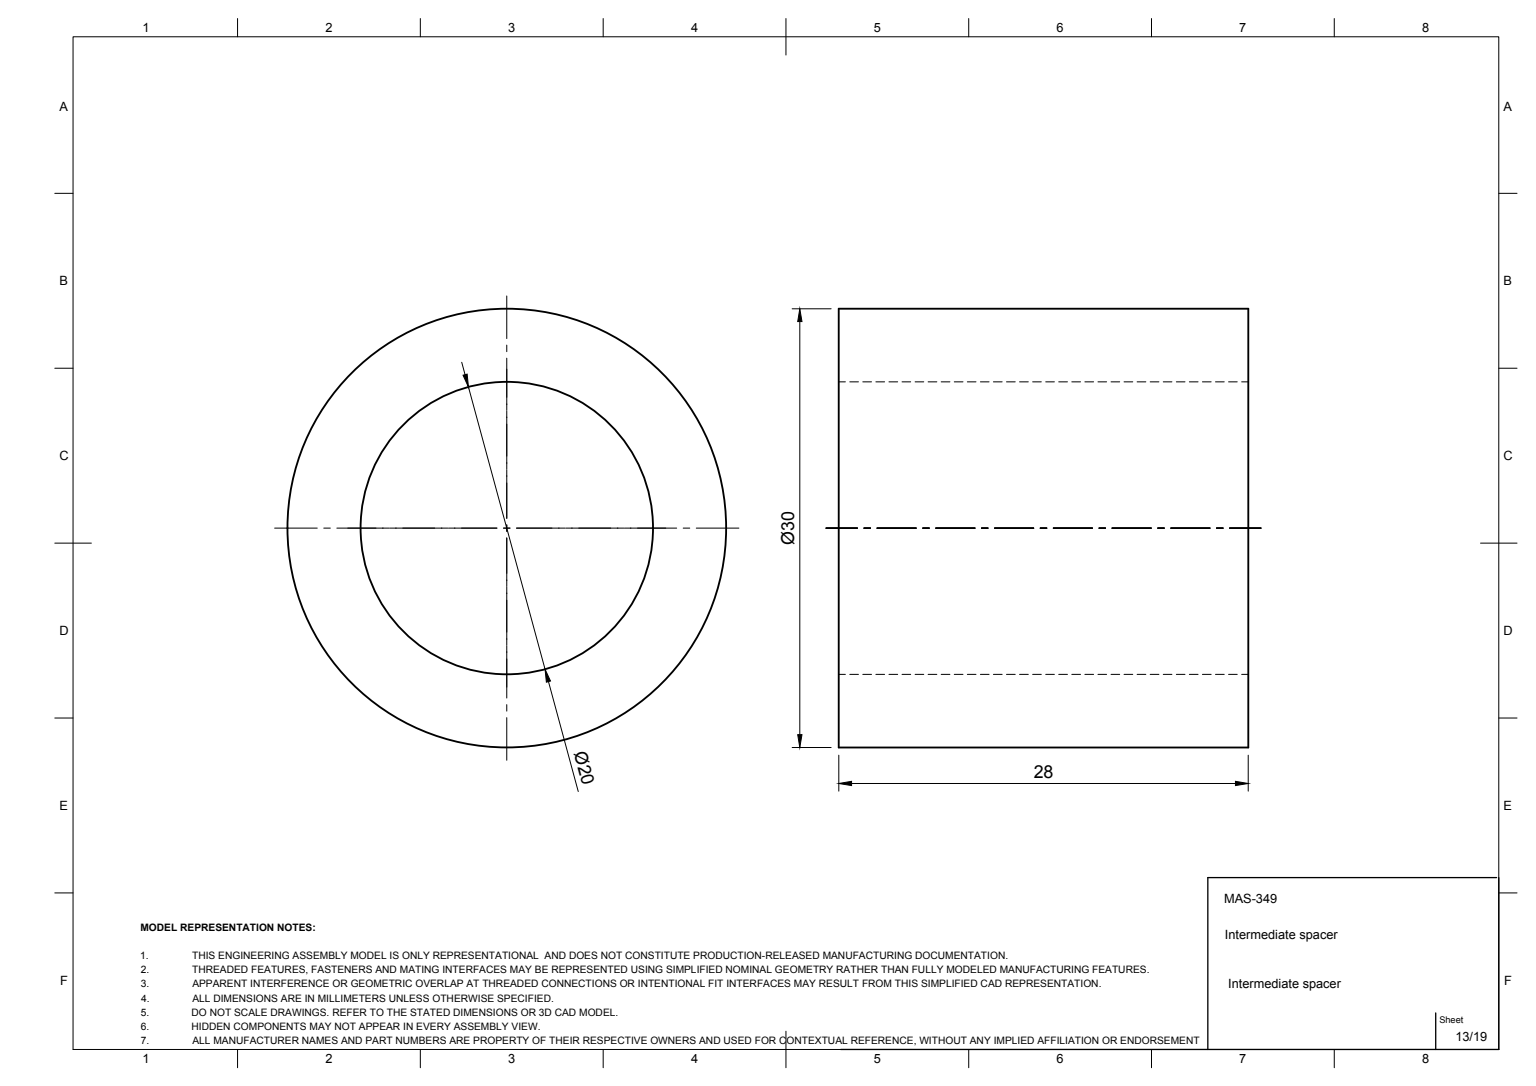
ISO-10303-21;
HEADER;
/* Generated by software containing ST-Developer
 * from STEP Tools, Inc. (www.steptools.com) 
 */

FILE_DESCRIPTION(
/* description */ ('Independent two-stage semi-open centrifugal-pump CAD. Shared impeller
s, open-machinable return casings, removable diaphragms, bronze wear/j
ournal rings, volume-preserving seal instances, retained keyed shaft, 
opposed mechanical face rings and partly threaded tie hardware. Native
 shaft rotation. Geometric topology/clearance only; flow/head/efficien
cy, pressure, cavitation, balance, preload, face loading and secondary
 seal fits/bonds, material/thermal/tolerance selection and life unassi
gned. External drive, coupling, anchors and piping bolts omitted.'),
/* implementation_level */ '2;1');

FILE_NAME(
/* name */ 'Intermediate spacer.step',
/* time_stamp */ '2026-11-08T18:06:32-08:00',
/* author */ (''),
/* organization */ (''),
/* preprocessor_version */ 'ST-DEVELOPER v20.2',
/* originating_system */ 'Autodesk Translation Framework v15.17.0.0',
/* authorisation */ '');

FILE_SCHEMA (('AUTOMOTIVE_DESIGN { 1 0 10303 214 3 1 1 }'));
ENDSEC;

DATA;
#10=MECHANICAL_DESIGN_GEOMETRIC_PRESENTATION_REPRESENTATION('',(#402),#16687);
#364=SHAPE_REPRESENTATION_RELATIONSHIP('SRR','None',#16773,#383);
#383=ADVANCED_BREP_SHAPE_REPRESENTATION('',(#421),#16677);
#402=STYLED_ITEM('',(#16874),#421);
#421=MANIFOLD_SOLID_BREP('Body1',#6121);
#537=FACE_BOUND('',#1418,.T.);
#538=FACE_BOUND('',#1420,.T.);
#653=PLANE('',#6840);
#654=PLANE('',#6841);
#962=FACE_OUTER_BOUND('',#1415,.T.);
#963=FACE_OUTER_BOUND('',#1416,.T.);
#964=FACE_OUTER_BOUND('',#1417,.T.);
#965=FACE_OUTER_BOUND('',#1419,.T.);
#1415=EDGE_LOOP('',(#5269,#5270,#5271,#5272));
#1416=EDGE_LOOP('',(#5273,#5274,#5275,#5276));
#1417=EDGE_LOOP('',(#5277));
#1418=EDGE_LOOP('',(#5278));
#1419=EDGE_LOOP('',(#5279));
#1420=EDGE_LOOP('',(#5280));
#1806=LINE('',#15120,#2175);
#1807=LINE('',#15126,#2176);
#2175=VECTOR('',#8282,1.);
#2176=VECTOR('',#8289,1.5);
#2454=CIRCLE('',#6835,1.);
#2455=CIRCLE('',#6836,1.);
#2456=CIRCLE('',#6838,1.5);
#2457=CIRCLE('',#6839,1.5);
#2957=VERTEX_POINT('',#15117);
#2958=VERTEX_POINT('',#15119);
#2959=VERTEX_POINT('',#15123);
#2960=VERTEX_POINT('',#15125);
#3744=EDGE_CURVE('',#2957,#2957,#2454,.T.);
#3745=EDGE_CURVE('',#2957,#2958,#1806,.T.);
#3746=EDGE_CURVE('',#2958,#2958,#2455,.T.);
#3747=EDGE_CURVE('',#2959,#2959,#2456,.T.);
#3748=EDGE_CURVE('',#2959,#2960,#1807,.T.);
#3749=EDGE_CURVE('',#2960,#2960,#2457,.T.);
#5269=ORIENTED_EDGE('',*,*,#3744,.F.);
#5270=ORIENTED_EDGE('',*,*,#3745,.T.);
#5271=ORIENTED_EDGE('',*,*,#3746,.T.);
#5272=ORIENTED_EDGE('',*,*,#3745,.F.);
#5273=ORIENTED_EDGE('',*,*,#3747,.F.);
#5274=ORIENTED_EDGE('',*,*,#3748,.T.);
#5275=ORIENTED_EDGE('',*,*,#3749,.T.);
#5276=ORIENTED_EDGE('',*,*,#3748,.F.);
#5277=ORIENTED_EDGE('',*,*,#3747,.T.);
#5278=ORIENTED_EDGE('',*,*,#3744,.T.);
#5279=ORIENTED_EDGE('',*,*,#3749,.F.);
#5280=ORIENTED_EDGE('',*,*,#3746,.F.);
#5730=CYLINDRICAL_SURFACE('',#6834,1.);
#5731=CYLINDRICAL_SURFACE('',#6837,1.5);
#6041=ADVANCED_FACE('',(#962),#5730,.F.);
#6042=ADVANCED_FACE('',(#963),#5731,.T.);
#6043=ADVANCED_FACE('',(#964,#537),#653,.T.);
#6044=ADVANCED_FACE('',(#965,#538),#654,.F.);
#6121=CLOSED_SHELL('',(#6041,#6042,#6043,#6044));
#6833=AXIS2_PLACEMENT_3D('',#15115,#8276,#8277);
#6834=AXIS2_PLACEMENT_3D('',#15116,#8278,#8279);
#6835=AXIS2_PLACEMENT_3D('',#15118,#8280,#8281);
#6836=AXIS2_PLACEMENT_3D('',#15121,#8283,#8284);
#6837=AXIS2_PLACEMENT_3D('',#15122,#8285,#8286);
#6838=AXIS2_PLACEMENT_3D('',#15124,#8287,#8288);
#6839=AXIS2_PLACEMENT_3D('',#15127,#8290,#8291);
#6840=AXIS2_PLACEMENT_3D('',#15128,#8292,#8293);
#6841=AXIS2_PLACEMENT_3D('',#15129,#8294,#8295);
#8276=DIRECTION('axis',(0.,0.,1.));
#8277=DIRECTION('refdir',(1.,0.,0.));
#8278=DIRECTION('center_axis',(0.,0.,1.));
#8279=DIRECTION('ref_axis',(1.,0.,0.));
#8280=DIRECTION('center_axis',(0.,0.,-1.));
#8281=DIRECTION('ref_axis',(1.,0.,0.));
#8282=DIRECTION('',(0.,0.,-1.));
#8283=DIRECTION('center_axis',(0.,0.,-1.));
#8284=DIRECTION('ref_axis',(1.,0.,0.));
#8285=DIRECTION('center_axis',(0.,0.,1.));
#8286=DIRECTION('ref_axis',(1.,0.,0.));
#8287=DIRECTION('center_axis',(0.,0.,1.));
#8288=DIRECTION('ref_axis',(1.,0.,0.));
#8289=DIRECTION('',(0.,0.,-1.));
#8290=DIRECTION('center_axis',(0.,0.,1.));
#8291=DIRECTION('ref_axis',(1.,0.,0.));
#8292=DIRECTION('center_axis',(0.,0.,1.));
#8293=DIRECTION('ref_axis',(1.,0.,0.));
#8294=DIRECTION('center_axis',(0.,0.,1.));
#8295=DIRECTION('ref_axis',(1.,0.,0.));
#15115=CARTESIAN_POINT('',(0.,0.,0.));
#15116=CARTESIAN_POINT('Origin',(0.,0.,3.2));
#15117=CARTESIAN_POINT('',(-1.,-1.22464679914735E-16,6.));
#15118=CARTESIAN_POINT('Origin',(0.,0.,6.));
#15119=CARTESIAN_POINT('',(-1.,-1.22464679914735E-16,3.2));
#15120=CARTESIAN_POINT('',(-1.,-1.22464679914735E-16,3.2));
#15121=CARTESIAN_POINT('Origin',(0.,0.,3.2));
#15122=CARTESIAN_POINT('Origin',(0.,0.,3.2));
#15123=CARTESIAN_POINT('',(-1.5,-1.83697019872103E-16,6.));
#15124=CARTESIAN_POINT('Origin',(0.,0.,6.));
#15125=CARTESIAN_POINT('',(-1.5,-1.83697019872103E-16,3.2));
#15126=CARTESIAN_POINT('',(-1.5,-1.83697019872103E-16,3.2));
#15127=CARTESIAN_POINT('Origin',(0.,0.,3.2));
#15128=CARTESIAN_POINT('Origin',(0.,0.,6.));
#15129=CARTESIAN_POINT('Origin',(0.,0.,3.2));
#16656=UNCERTAINTY_MEASURE_WITH_UNIT(LENGTH_MEASURE(0.001),#16688,
'DISTANCE_ACCURACY_VALUE',
'Maximum model space distance between geometric entities at asserted c
onnectivities');
#16666=UNCERTAINTY_MEASURE_WITH_UNIT(LENGTH_MEASURE(0.001),#16688,
'DISTANCE_ACCURACY_VALUE',
'Maximum model space distance between geometric entities at asserted c
onnectivities');
#16677=(
GEOMETRIC_REPRESENTATION_CONTEXT(3)
GLOBAL_UNCERTAINTY_ASSIGNED_CONTEXT((#16656))
GLOBAL_UNIT_ASSIGNED_CONTEXT((#16688,#16690,#16691))
REPRESENTATION_CONTEXT('','3D')
);
#16687=(
GEOMETRIC_REPRESENTATION_CONTEXT(3)
GLOBAL_UNCERTAINTY_ASSIGNED_CONTEXT((#16666))
GLOBAL_UNIT_ASSIGNED_CONTEXT((#16688,#16690,#16691))
REPRESENTATION_CONTEXT('','3D')
);
#16688=(
LENGTH_UNIT()
NAMED_UNIT(*)
SI_UNIT(.CENTI.,.METRE.)
);
#16690=(
NAMED_UNIT(*)
PLANE_ANGLE_UNIT()
SI_UNIT($,.RADIAN.)
);
#16691=(
NAMED_UNIT(*)
SI_UNIT($,.STERADIAN.)
SOLID_ANGLE_UNIT()
);
#16702=SHAPE_DEFINITION_REPRESENTATION(#16722,#16773);
#16722=PRODUCT_DEFINITION_SHAPE('',$,#16794);
#16773=SHAPE_REPRESENTATION('',(#6833),#16677);
#16783=PRODUCT_DEFINITION_CONTEXT('part definition',#16845,'design');
#16794=PRODUCT_DEFINITION('Intermediate spacer','Intermediate spacer',#16814,
#16783);
#16814=PRODUCT_DEFINITION_FORMATION('',$,#16857);
#16845=APPLICATION_CONTEXT(
'Core Data for Automotive Mechanical Design Process');
#16846=PRODUCT_CONTEXT('part definition',#16845,'mechanical');
#16857=PRODUCT('Intermediate spacer','Intermediate spacer',$,(#16846));
#16874=PRESENTATION_STYLE_ASSIGNMENT((#16889));
#16889=SURFACE_STYLE_USAGE(.BOTH.,#16904);
#16904=SURFACE_SIDE_STYLE('',(#16919));
#16919=SURFACE_STYLE_FILL_AREA(#16934);
#16934=FILL_AREA_STYLE('Spacer gray',(#16949));
#16949=FILL_AREA_STYLE_COLOUR('Spacer gray',#16964);
#16964=COLOUR_RGB('Spacer gray',0.576470588235294,0.615686274509804,0.666666666666667);
ENDSEC;
END-ISO-10303-21;
